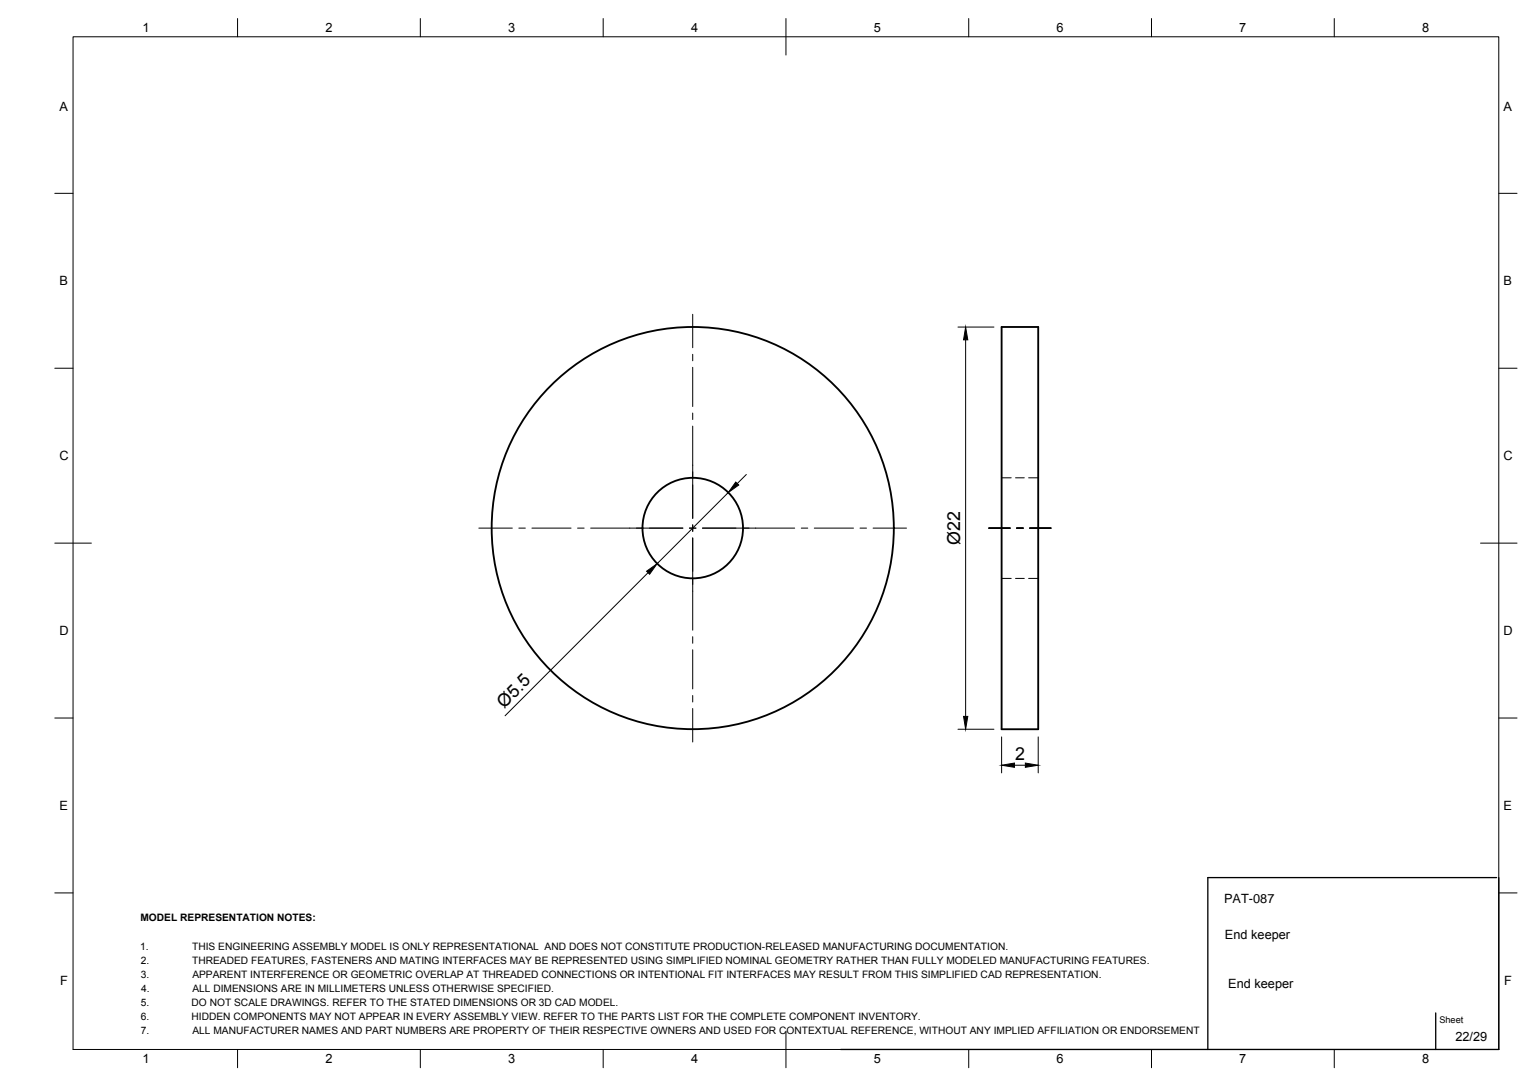
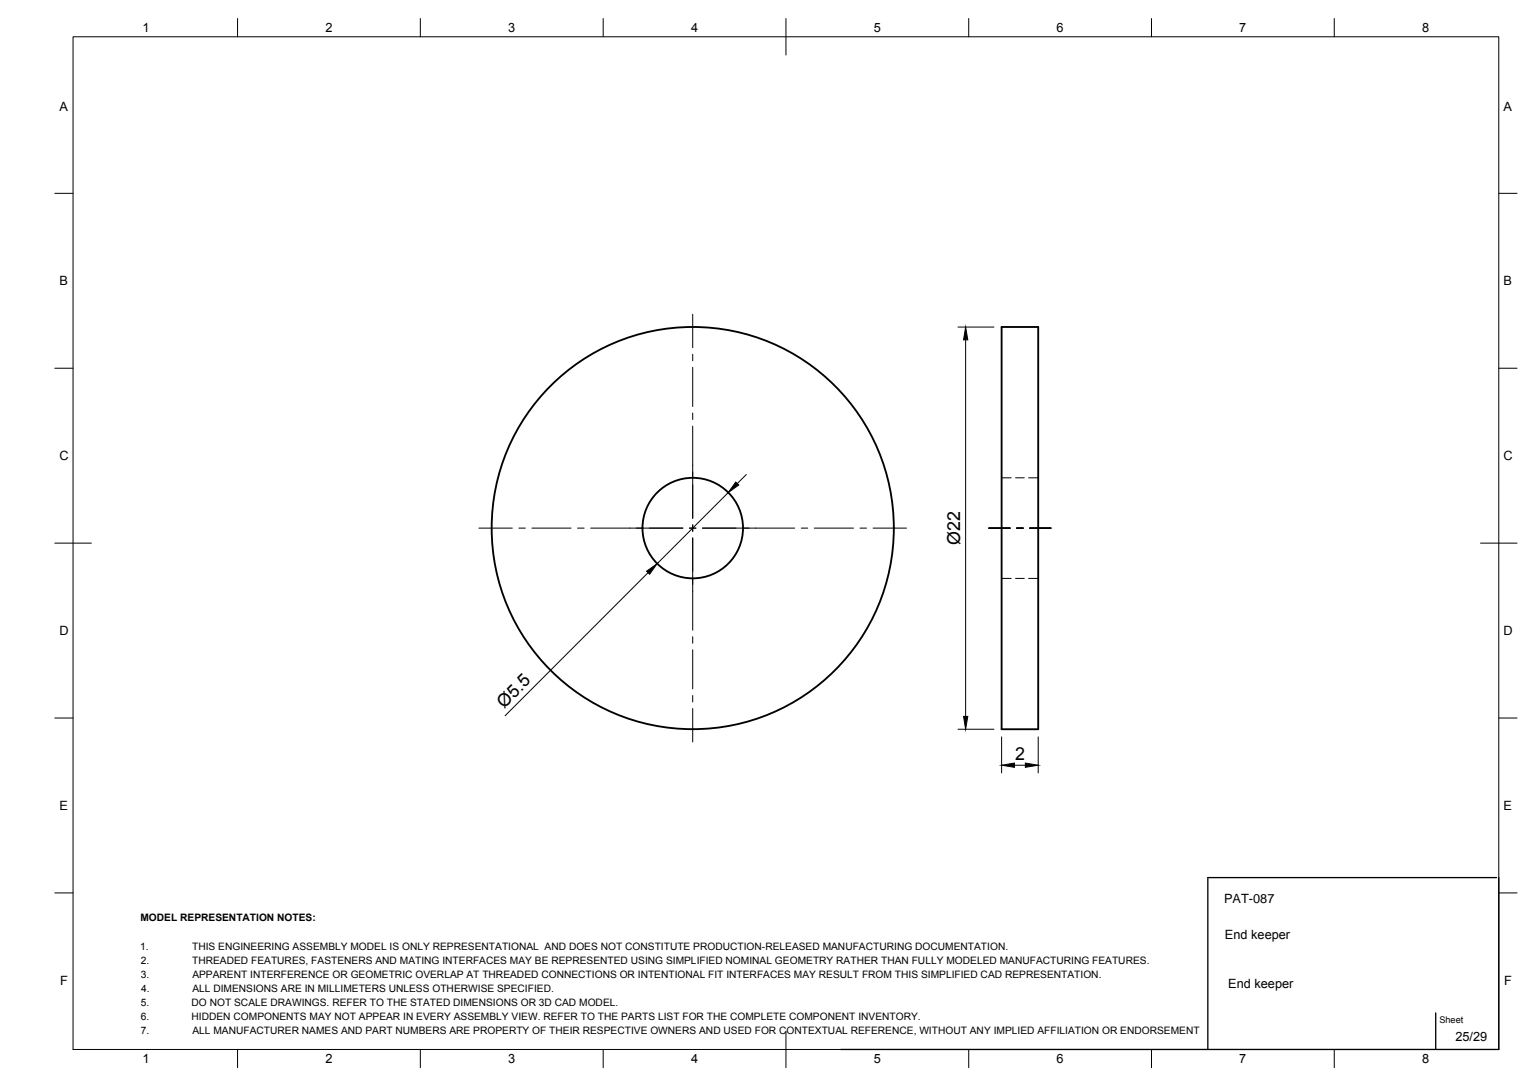
ISO-10303-21;
HEADER;
/* Generated by software containing ST-Developer
 * from STEP Tools, Inc. (www.steptools.com) 
 */

FILE_DESCRIPTION(
/* description */ ('Rigid flange shaft coupling assembly'),
/* implementation_level */ '2;1');

FILE_NAME(
/* name */ 'End keeper.step',
/* time_stamp */ '2026-10-27T10:47:16-07:00',
/* author */ (''),
/* organization */ (''),
/* preprocessor_version */ 'ST-DEVELOPER v20.2',
/* originating_system */ 'Autodesk Translation Framework v15.17.0.0',
/* authorisation */ '');

FILE_SCHEMA (('AUTOMOTIVE_DESIGN { 1 0 10303 214 3 1 1 }'));
ENDSEC;

DATA;
#10=MECHANICAL_DESIGN_GEOMETRIC_PRESENTATION_REPRESENTATION('',(#414),#9141);
#357=SHAPE_REPRESENTATION_RELATIONSHIP('SRR','None',#9293,#385);
#385=ADVANCED_BREP_SHAPE_REPRESENTATION('',(#442),#9128);
#414=STYLED_ITEM('',(#9514),#442);
#442=MANIFOLD_SOLID_BREP('Body1',#4769);
#533=FACE_BOUND('',#1246,.T.);
#534=FACE_BOUND('',#1248,.T.);
#662=PLANE('',#5370);
#663=PLANE('',#5371);
#891=FACE_OUTER_BOUND('',#1243,.T.);
#892=FACE_OUTER_BOUND('',#1244,.T.);
#893=FACE_OUTER_BOUND('',#1245,.T.);
#894=FACE_OUTER_BOUND('',#1247,.T.);
#1243=EDGE_LOOP('',(#3889,#3890,#3891,#3892));
#1244=EDGE_LOOP('',(#3893,#3894,#3895,#3896));
#1245=EDGE_LOOP('',(#3897));
#1246=EDGE_LOOP('',(#3898));
#1247=EDGE_LOOP('',(#3899));
#1248=EDGE_LOOP('',(#3900));
#1598=LINE('',#8263,#1943);
#1599=LINE('',#8269,#1944);
#1943=VECTOR('',#6381,0.275);
#1944=VECTOR('',#6388,1.1);
#2197=CIRCLE('',#5365,0.275);
#2198=CIRCLE('',#5366,0.275);
#2199=CIRCLE('',#5368,1.1);
#2200=CIRCLE('',#5369,1.1);
#2498=VERTEX_POINT('',#8260);
#2499=VERTEX_POINT('',#8262);
#2500=VERTEX_POINT('',#8266);
#2501=VERTEX_POINT('',#8268);
#2988=EDGE_CURVE('',#2498,#2498,#2197,.T.);
#2989=EDGE_CURVE('',#2498,#2499,#1598,.T.);
#2990=EDGE_CURVE('',#2499,#2499,#2198,.T.);
#2991=EDGE_CURVE('',#2500,#2500,#2199,.T.);
#2992=EDGE_CURVE('',#2500,#2501,#1599,.T.);
#2993=EDGE_CURVE('',#2501,#2501,#2200,.T.);
#3889=ORIENTED_EDGE('',*,*,#2988,.F.);
#3890=ORIENTED_EDGE('',*,*,#2989,.T.);
#3891=ORIENTED_EDGE('',*,*,#2990,.T.);
#3892=ORIENTED_EDGE('',*,*,#2989,.F.);
#3893=ORIENTED_EDGE('',*,*,#2991,.F.);
#3894=ORIENTED_EDGE('',*,*,#2992,.T.);
#3895=ORIENTED_EDGE('',*,*,#2993,.T.);
#3896=ORIENTED_EDGE('',*,*,#2992,.F.);
#3897=ORIENTED_EDGE('',*,*,#2991,.T.);
#3898=ORIENTED_EDGE('',*,*,#2988,.T.);
#3899=ORIENTED_EDGE('',*,*,#2993,.F.);
#3900=ORIENTED_EDGE('',*,*,#2990,.F.);
#4449=CYLINDRICAL_SURFACE('',#5364,0.275);
#4450=CYLINDRICAL_SURFACE('',#5367,1.1);
#4627=ADVANCED_FACE('',(#891),#4449,.F.);
#4628=ADVANCED_FACE('',(#892),#4450,.T.);
#4629=ADVANCED_FACE('',(#893,#533),#662,.T.);
#4630=ADVANCED_FACE('',(#894,#534),#663,.F.);
#4769=CLOSED_SHELL('',(#4627,#4628,#4629,#4630));
#5363=AXIS2_PLACEMENT_3D('',#8258,#6375,#6376);
#5364=AXIS2_PLACEMENT_3D('',#8259,#6377,#6378);
#5365=AXIS2_PLACEMENT_3D('',#8261,#6379,#6380);
#5366=AXIS2_PLACEMENT_3D('',#8264,#6382,#6383);
#5367=AXIS2_PLACEMENT_3D('',#8265,#6384,#6385);
#5368=AXIS2_PLACEMENT_3D('',#8267,#6386,#6387);
#5369=AXIS2_PLACEMENT_3D('',#8270,#6389,#6390);
#5370=AXIS2_PLACEMENT_3D('',#8271,#6391,#6392);
#5371=AXIS2_PLACEMENT_3D('',#8272,#6393,#6394);
#6375=DIRECTION('axis',(0.,0.,1.));
#6376=DIRECTION('refdir',(1.,0.,0.));
#6377=DIRECTION('center_axis',(0.,1.,0.));
#6378=DIRECTION('ref_axis',(1.,0.,0.));
#6379=DIRECTION('center_axis',(0.,-1.,0.));
#6380=DIRECTION('ref_axis',(1.,0.,0.));
#6381=DIRECTION('',(0.,-1.,0.));
#6382=DIRECTION('center_axis',(0.,-1.,0.));
#6383=DIRECTION('ref_axis',(1.,0.,0.));
#6384=DIRECTION('center_axis',(0.,1.,0.));
#6385=DIRECTION('ref_axis',(1.,0.,0.));
#6386=DIRECTION('center_axis',(0.,1.,0.));
#6387=DIRECTION('ref_axis',(1.,0.,0.));
#6388=DIRECTION('',(0.,-1.,0.));
#6389=DIRECTION('center_axis',(0.,1.,0.));
#6390=DIRECTION('ref_axis',(1.,0.,0.));
#6391=DIRECTION('center_axis',(0.,1.,0.));
#6392=DIRECTION('ref_axis',(1.,0.,0.));
#6393=DIRECTION('center_axis',(0.,1.,0.));
#6394=DIRECTION('ref_axis',(1.,0.,0.));
#8258=CARTESIAN_POINT('',(0.,0.,0.));
#8259=CARTESIAN_POINT('Origin',(0.,-4.7,6.53));
#8260=CARTESIAN_POINT('',(-0.275,-4.5,6.53));
#8261=CARTESIAN_POINT('Origin',(0.,-4.5,6.53));
#8262=CARTESIAN_POINT('',(-0.275,-4.7,6.53));
#8263=CARTESIAN_POINT('',(-0.275,-4.7,6.53));
#8264=CARTESIAN_POINT('Origin',(0.,-4.7,6.53));
#8265=CARTESIAN_POINT('Origin',(0.,-4.7,6.53));
#8266=CARTESIAN_POINT('',(-1.1,-4.5,6.53));
#8267=CARTESIAN_POINT('Origin',(0.,-4.5,6.53));
#8268=CARTESIAN_POINT('',(-1.1,-4.7,6.53));
#8269=CARTESIAN_POINT('',(-1.1,-4.7,6.53));
#8270=CARTESIAN_POINT('Origin',(0.,-4.7,6.53));
#8271=CARTESIAN_POINT('Origin',(0.,-4.5,6.53));
#8272=CARTESIAN_POINT('Origin',(0.,-4.7,6.53));
#9095=UNCERTAINTY_MEASURE_WITH_UNIT(LENGTH_MEASURE(0.001),#9142,
'DISTANCE_ACCURACY_VALUE',
'Maximum model space distance between geometric entities at asserted c
onnectivities');
#9108=UNCERTAINTY_MEASURE_WITH_UNIT(LENGTH_MEASURE(0.001),#9142,
'DISTANCE_ACCURACY_VALUE',
'Maximum model space distance between geometric entities at asserted c
onnectivities');
#9128=(
GEOMETRIC_REPRESENTATION_CONTEXT(3)
GLOBAL_UNCERTAINTY_ASSIGNED_CONTEXT((#9095))
GLOBAL_UNIT_ASSIGNED_CONTEXT((#9142,#9144,#9145))
REPRESENTATION_CONTEXT('','3D')
);
#9141=(
GEOMETRIC_REPRESENTATION_CONTEXT(3)
GLOBAL_UNCERTAINTY_ASSIGNED_CONTEXT((#9108))
GLOBAL_UNIT_ASSIGNED_CONTEXT((#9142,#9144,#9145))
REPRESENTATION_CONTEXT('','3D')
);
#9142=(
LENGTH_UNIT()
NAMED_UNIT(*)
SI_UNIT(.CENTI.,.METRE.)
);
#9144=(
NAMED_UNIT(*)
PLANE_ANGLE_UNIT()
SI_UNIT($,.RADIAN.)
);
#9145=(
NAMED_UNIT(*)
SI_UNIT($,.STERADIAN.)
SOLID_ANGLE_UNIT()
);
#9165=SHAPE_DEFINITION_REPRESENTATION(#9199,#9293);
#9199=PRODUCT_DEFINITION_SHAPE('',$,#9326);
#9293=SHAPE_REPRESENTATION('',(#5363),#9128);
#9306=PRODUCT_DEFINITION_CONTEXT('part definition',#9404,'design');
#9326=PRODUCT_DEFINITION('End keeper','End keeper',#9358,#9306);
#9358=PRODUCT_DEFINITION_FORMATION('',$,#9425);
#9404=APPLICATION_CONTEXT(
'Core Data for Automotive Mechanical Design Process');
#9405=PRODUCT_CONTEXT('part definition',#9404,'mechanical');
#9425=PRODUCT('End keeper','End keeper','End keeper',(#9405));
#9508=COLOUR_RGB('Off White',0.89,0.88,0.83);
#9509=FILL_AREA_STYLE_COLOUR('',#9508);
#9510=FILL_AREA_STYLE('',(#9509));
#9511=SURFACE_STYLE_FILL_AREA(#9510);
#9512=SURFACE_SIDE_STYLE('',(#9511));
#9513=SURFACE_STYLE_USAGE(.BOTH.,#9512);
#9514=PRESENTATION_STYLE_ASSIGNMENT((#9513));
ENDSEC;
END-ISO-10303-21;
